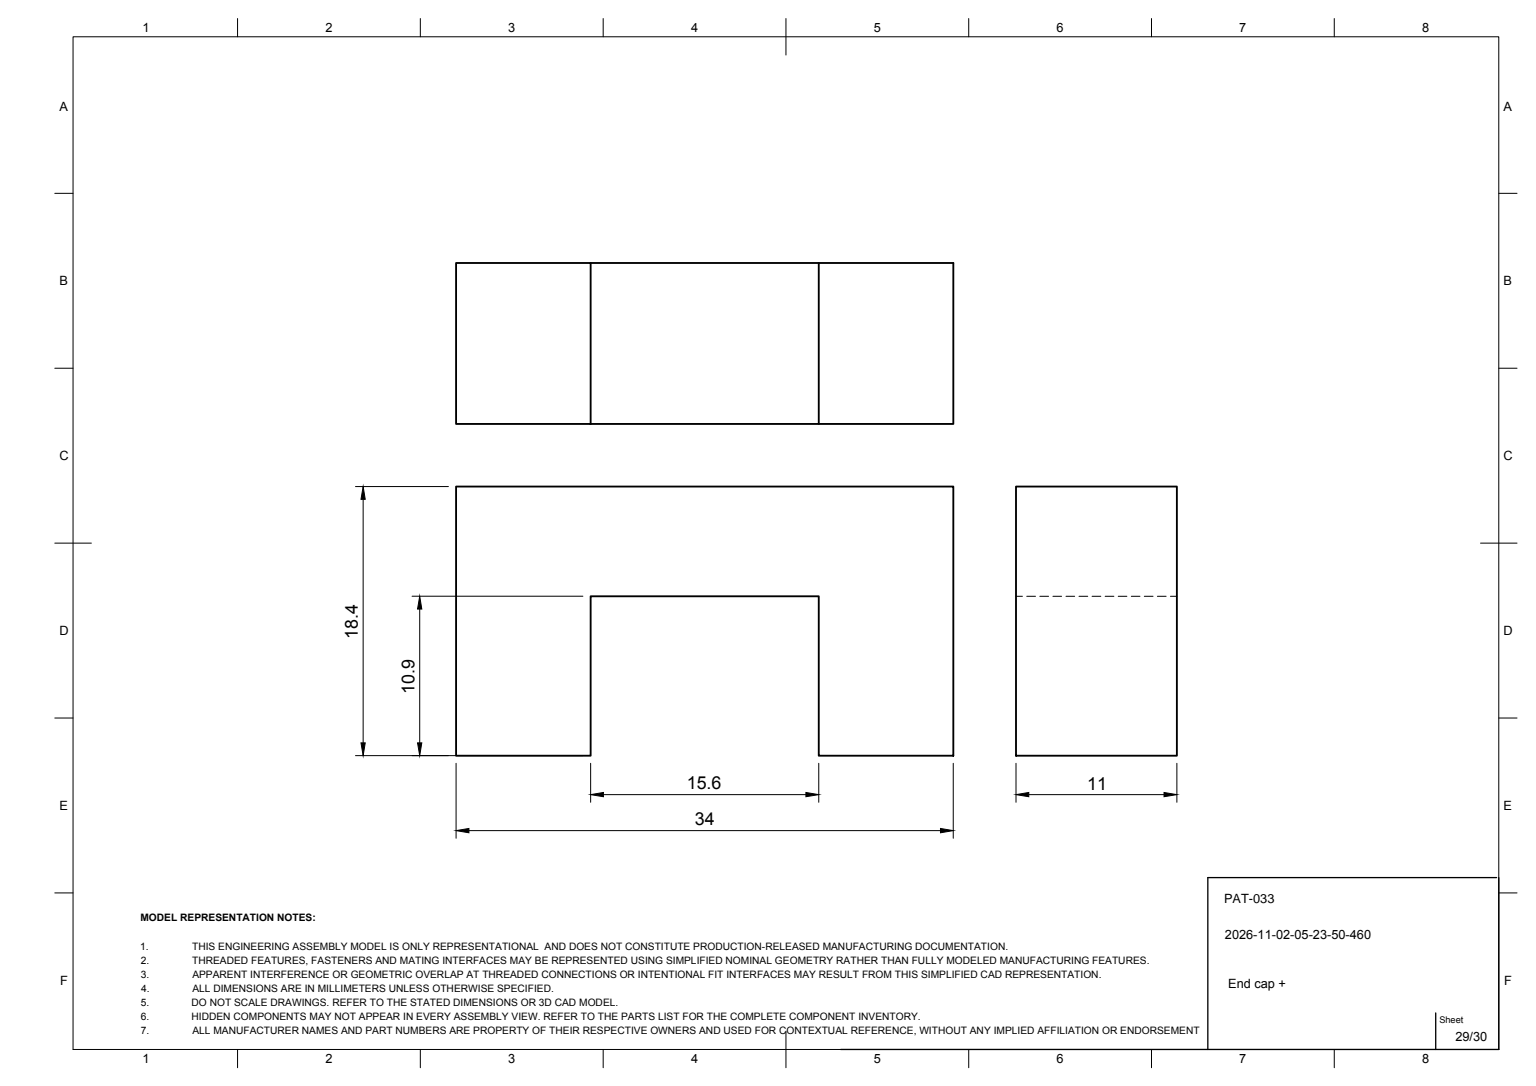
ISO-10303-21;
HEADER;
/* Generated by software containing ST-Developer
 * from STEP Tools, Inc. (www.steptools.com) 
 */

FILE_DESCRIPTION(
/* description */ ('Dual-rail gantry carriage'),
/* implementation_level */ '2;1');

FILE_NAME(
/* name */ 'End cap +.step',
/* time_stamp */ '2026-10-27T10:49:15-07:00',
/* author */ (''),
/* organization */ (''),
/* preprocessor_version */ 'ST-DEVELOPER v20.2',
/* originating_system */ 'Autodesk Translation Framework v15.17.0.0',
/* authorisation */ '');

FILE_SCHEMA (('AUTOMOTIVE_DESIGN { 1 0 10303 214 3 1 1 }'));
ENDSEC;

DATA;
#10=MECHANICAL_DESIGN_GEOMETRIC_PRESENTATION_REPRESENTATION('',(#608),#12804);
#546=SHAPE_REPRESENTATION_RELATIONSHIP('SRR','None',#13026,#577);
#577=ADVANCED_BREP_SHAPE_REPRESENTATION('',(#637),#12796);
#608=STYLED_ITEM('',(#13240),#637);
#637=MANIFOLD_SOLID_BREP('Body1',#7388);
#989=PLANE('',#8239);
#990=PLANE('',#8240);
#991=PLANE('',#8241);
#992=PLANE('',#8242);
#993=PLANE('',#8243);
#994=PLANE('',#8244);
#995=PLANE('',#8245);
#996=PLANE('',#8246);
#997=PLANE('',#8247);
#998=PLANE('',#8248);
#1353=FACE_OUTER_BOUND('',#1855,.T.);
#1354=FACE_OUTER_BOUND('',#1856,.T.);
#1355=FACE_OUTER_BOUND('',#1857,.T.);
#1356=FACE_OUTER_BOUND('',#1858,.T.);
#1357=FACE_OUTER_BOUND('',#1859,.T.);
#1358=FACE_OUTER_BOUND('',#1860,.T.);
#1359=FACE_OUTER_BOUND('',#1861,.T.);
#1360=FACE_OUTER_BOUND('',#1862,.T.);
#1361=FACE_OUTER_BOUND('',#1863,.T.);
#1362=FACE_OUTER_BOUND('',#1864,.T.);
#1855=EDGE_LOOP('',(#6561,#6562,#6563,#6564));
#1856=EDGE_LOOP('',(#6565,#6566,#6567,#6568));
#1857=EDGE_LOOP('',(#6569,#6570,#6571,#6572));
#1858=EDGE_LOOP('',(#6573,#6574,#6575,#6576));
#1859=EDGE_LOOP('',(#6577,#6578,#6579,#6580));
#1860=EDGE_LOOP('',(#6581,#6582,#6583,#6584));
#1861=EDGE_LOOP('',(#6585,#6586,#6587,#6588));
#1862=EDGE_LOOP('',(#6589,#6590,#6591,#6592));
#1863=EDGE_LOOP('',(#6593,#6594,#6595,#6596,#6597,#6598,#6599,#6600));
#1864=EDGE_LOOP('',(#6601,#6602,#6603,#6604,#6605,#6606,#6607,#6608));
#2530=LINE('',#12256,#3239);
#2531=LINE('',#12258,#3240);
#2532=LINE('',#12260,#3241);
#2533=LINE('',#12261,#3242);
#2534=LINE('',#12264,#3243);
#2535=LINE('',#12266,#3244);
#2536=LINE('',#12267,#3245);
#2537=LINE('',#12270,#3246);
#2538=LINE('',#12272,#3247);
#2539=LINE('',#12273,#3248);
#2540=LINE('',#12276,#3249);
#2541=LINE('',#12278,#3250);
#2542=LINE('',#12279,#3251);
#2543=LINE('',#12282,#3252);
#2544=LINE('',#12284,#3253);
#2545=LINE('',#12285,#3254);
#2546=LINE('',#12288,#3255);
#2547=LINE('',#12290,#3256);
#2548=LINE('',#12291,#3257);
#2549=LINE('',#12294,#3258);
#2550=LINE('',#12296,#3259);
#2551=LINE('',#12297,#3260);
#2552=LINE('',#12299,#3261);
#2553=LINE('',#12300,#3262);
#3239=VECTOR('',#10067,1.);
#3240=VECTOR('',#10068,1.);
#3241=VECTOR('',#10069,1.);
#3242=VECTOR('',#10070,1.);
#3243=VECTOR('',#10073,1.);
#3244=VECTOR('',#10074,1.);
#3245=VECTOR('',#10075,1.);
#3246=VECTOR('',#10078,1.);
#3247=VECTOR('',#10079,1.);
#3248=VECTOR('',#10080,1.);
#3249=VECTOR('',#10083,1.);
#3250=VECTOR('',#10084,1.);
#3251=VECTOR('',#10085,1.);
#3252=VECTOR('',#10088,1.);
#3253=VECTOR('',#10089,1.);
#3254=VECTOR('',#10090,1.);
#3255=VECTOR('',#10093,1.);
#3256=VECTOR('',#10094,1.);
#3257=VECTOR('',#10095,1.);
#3258=VECTOR('',#10098,1.);
#3259=VECTOR('',#10099,1.);
#3260=VECTOR('',#10100,1.);
#3261=VECTOR('',#10103,1.);
#3262=VECTOR('',#10104,1.);
#4051=VERTEX_POINT('',#12254);
#4052=VERTEX_POINT('',#12255);
#4053=VERTEX_POINT('',#12257);
#4054=VERTEX_POINT('',#12259);
#4055=VERTEX_POINT('',#12263);
#4056=VERTEX_POINT('',#12265);
#4057=VERTEX_POINT('',#12269);
#4058=VERTEX_POINT('',#12271);
#4059=VERTEX_POINT('',#12275);
#4060=VERTEX_POINT('',#12277);
#4061=VERTEX_POINT('',#12281);
#4062=VERTEX_POINT('',#12283);
#4063=VERTEX_POINT('',#12287);
#4064=VERTEX_POINT('',#12289);
#4065=VERTEX_POINT('',#12293);
#4066=VERTEX_POINT('',#12295);
#4903=EDGE_CURVE('',#4051,#4052,#2530,.T.);
#4904=EDGE_CURVE('',#4052,#4053,#2531,.T.);
#4905=EDGE_CURVE('',#4054,#4053,#2532,.T.);
#4906=EDGE_CURVE('',#4051,#4054,#2533,.T.);
#4907=EDGE_CURVE('',#4055,#4051,#2534,.T.);
#4908=EDGE_CURVE('',#4056,#4054,#2535,.T.);
#4909=EDGE_CURVE('',#4055,#4056,#2536,.T.);
#4910=EDGE_CURVE('',#4057,#4055,#2537,.T.);
#4911=EDGE_CURVE('',#4058,#4056,#2538,.T.);
#4912=EDGE_CURVE('',#4057,#4058,#2539,.T.);
#4913=EDGE_CURVE('',#4059,#4057,#2540,.T.);
#4914=EDGE_CURVE('',#4060,#4058,#2541,.T.);
#4915=EDGE_CURVE('',#4059,#4060,#2542,.T.);
#4916=EDGE_CURVE('',#4061,#4059,#2543,.T.);
#4917=EDGE_CURVE('',#4062,#4060,#2544,.T.);
#4918=EDGE_CURVE('',#4061,#4062,#2545,.T.);
#4919=EDGE_CURVE('',#4063,#4061,#2546,.T.);
#4920=EDGE_CURVE('',#4064,#4062,#2547,.T.);
#4921=EDGE_CURVE('',#4063,#4064,#2548,.T.);
#4922=EDGE_CURVE('',#4065,#4063,#2549,.T.);
#4923=EDGE_CURVE('',#4066,#4064,#2550,.T.);
#4924=EDGE_CURVE('',#4065,#4066,#2551,.T.);
#4925=EDGE_CURVE('',#4052,#4065,#2552,.T.);
#4926=EDGE_CURVE('',#4053,#4066,#2553,.T.);
#6561=ORIENTED_EDGE('',*,*,#4903,.T.);
#6562=ORIENTED_EDGE('',*,*,#4904,.T.);
#6563=ORIENTED_EDGE('',*,*,#4905,.F.);
#6564=ORIENTED_EDGE('',*,*,#4906,.F.);
#6565=ORIENTED_EDGE('',*,*,#4907,.T.);
#6566=ORIENTED_EDGE('',*,*,#4906,.T.);
#6567=ORIENTED_EDGE('',*,*,#4908,.F.);
#6568=ORIENTED_EDGE('',*,*,#4909,.F.);
#6569=ORIENTED_EDGE('',*,*,#4910,.T.);
#6570=ORIENTED_EDGE('',*,*,#4909,.T.);
#6571=ORIENTED_EDGE('',*,*,#4911,.F.);
#6572=ORIENTED_EDGE('',*,*,#4912,.F.);
#6573=ORIENTED_EDGE('',*,*,#4913,.T.);
#6574=ORIENTED_EDGE('',*,*,#4912,.T.);
#6575=ORIENTED_EDGE('',*,*,#4914,.F.);
#6576=ORIENTED_EDGE('',*,*,#4915,.F.);
#6577=ORIENTED_EDGE('',*,*,#4916,.T.);
#6578=ORIENTED_EDGE('',*,*,#4915,.T.);
#6579=ORIENTED_EDGE('',*,*,#4917,.F.);
#6580=ORIENTED_EDGE('',*,*,#4918,.F.);
#6581=ORIENTED_EDGE('',*,*,#4919,.T.);
#6582=ORIENTED_EDGE('',*,*,#4918,.T.);
#6583=ORIENTED_EDGE('',*,*,#4920,.F.);
#6584=ORIENTED_EDGE('',*,*,#4921,.F.);
#6585=ORIENTED_EDGE('',*,*,#4922,.T.);
#6586=ORIENTED_EDGE('',*,*,#4921,.T.);
#6587=ORIENTED_EDGE('',*,*,#4923,.F.);
#6588=ORIENTED_EDGE('',*,*,#4924,.F.);
#6589=ORIENTED_EDGE('',*,*,#4925,.T.);
#6590=ORIENTED_EDGE('',*,*,#4924,.T.);
#6591=ORIENTED_EDGE('',*,*,#4926,.F.);
#6592=ORIENTED_EDGE('',*,*,#4904,.F.);
#6593=ORIENTED_EDGE('',*,*,#4926,.T.);
#6594=ORIENTED_EDGE('',*,*,#4923,.T.);
#6595=ORIENTED_EDGE('',*,*,#4920,.T.);
#6596=ORIENTED_EDGE('',*,*,#4917,.T.);
#6597=ORIENTED_EDGE('',*,*,#4914,.T.);
#6598=ORIENTED_EDGE('',*,*,#4911,.T.);
#6599=ORIENTED_EDGE('',*,*,#4908,.T.);
#6600=ORIENTED_EDGE('',*,*,#4905,.T.);
#6601=ORIENTED_EDGE('',*,*,#4925,.F.);
#6602=ORIENTED_EDGE('',*,*,#4903,.F.);
#6603=ORIENTED_EDGE('',*,*,#4907,.F.);
#6604=ORIENTED_EDGE('',*,*,#4910,.F.);
#6605=ORIENTED_EDGE('',*,*,#4913,.F.);
#6606=ORIENTED_EDGE('',*,*,#4916,.F.);
#6607=ORIENTED_EDGE('',*,*,#4919,.F.);
#6608=ORIENTED_EDGE('',*,*,#4922,.F.);
#7279=ADVANCED_FACE('',(#1353),#989,.T.);
#7280=ADVANCED_FACE('',(#1354),#990,.T.);
#7281=ADVANCED_FACE('',(#1355),#991,.T.);
#7282=ADVANCED_FACE('',(#1356),#992,.T.);
#7283=ADVANCED_FACE('',(#1357),#993,.T.);
#7284=ADVANCED_FACE('',(#1358),#994,.T.);
#7285=ADVANCED_FACE('',(#1359),#995,.T.);
#7286=ADVANCED_FACE('',(#1360),#996,.T.);
#7287=ADVANCED_FACE('',(#1361),#997,.T.);
#7288=ADVANCED_FACE('',(#1362),#998,.F.);
#7388=CLOSED_SHELL('',(#7279,#7280,#7281,#7282,#7283,#7284,#7285,#7286,
#7287,#7288));
#8238=AXIS2_PLACEMENT_3D('',#12252,#10063,#10064);
#8239=AXIS2_PLACEMENT_3D('',#12253,#10065,#10066);
#8240=AXIS2_PLACEMENT_3D('',#12262,#10071,#10072);
#8241=AXIS2_PLACEMENT_3D('',#12268,#10076,#10077);
#8242=AXIS2_PLACEMENT_3D('',#12274,#10081,#10082);
#8243=AXIS2_PLACEMENT_3D('',#12280,#10086,#10087);
#8244=AXIS2_PLACEMENT_3D('',#12286,#10091,#10092);
#8245=AXIS2_PLACEMENT_3D('',#12292,#10096,#10097);
#8246=AXIS2_PLACEMENT_3D('',#12298,#10101,#10102);
#8247=AXIS2_PLACEMENT_3D('',#12301,#10105,#10106);
#8248=AXIS2_PLACEMENT_3D('',#12302,#10107,#10108);
#10063=DIRECTION('axis',(0.,0.,1.));
#10064=DIRECTION('refdir',(1.,0.,0.));
#10065=DIRECTION('center_axis',(0.,0.,1.));
#10066=DIRECTION('ref_axis',(0.,-1.,0.));
#10067=DIRECTION('',(0.,-1.,0.));
#10068=DIRECTION('',(1.,0.,0.));
#10069=DIRECTION('',(0.,-1.,0.));
#10070=DIRECTION('',(1.,0.,0.));
#10071=DIRECTION('center_axis',(0.,1.,0.));
#10072=DIRECTION('ref_axis',(0.,0.,1.));
#10073=DIRECTION('',(0.,0.,1.));
#10074=DIRECTION('',(0.,0.,1.));
#10075=DIRECTION('',(1.,0.,0.));
#10076=DIRECTION('center_axis',(0.,0.,-1.));
#10077=DIRECTION('ref_axis',(0.,1.,0.));
#10078=DIRECTION('',(0.,1.,0.));
#10079=DIRECTION('',(0.,1.,0.));
#10080=DIRECTION('',(1.,0.,0.));
#10081=DIRECTION('center_axis',(0.,-1.,0.));
#10082=DIRECTION('ref_axis',(0.,0.,-1.));
#10083=DIRECTION('',(0.,0.,-1.));
#10084=DIRECTION('',(0.,0.,-1.));
#10085=DIRECTION('',(1.,0.,0.));
#10086=DIRECTION('center_axis',(0.,0.,-1.));
#10087=DIRECTION('ref_axis',(0.,1.,0.));
#10088=DIRECTION('',(0.,1.,0.));
#10089=DIRECTION('',(0.,1.,0.));
#10090=DIRECTION('',(1.,0.,0.));
#10091=DIRECTION('center_axis',(0.,1.,0.));
#10092=DIRECTION('ref_axis',(0.,0.,1.));
#10093=DIRECTION('',(0.,0.,1.));
#10094=DIRECTION('',(0.,0.,1.));
#10095=DIRECTION('',(1.,0.,0.));
#10096=DIRECTION('center_axis',(0.,0.,-1.));
#10097=DIRECTION('ref_axis',(0.,1.,0.));
#10098=DIRECTION('',(0.,1.,0.));
#10099=DIRECTION('',(0.,1.,0.));
#10100=DIRECTION('',(1.,0.,0.));
#10101=DIRECTION('center_axis',(0.,-1.,0.));
#10102=DIRECTION('ref_axis',(0.,0.,-1.));
#10103=DIRECTION('',(0.,0.,-1.));
#10104=DIRECTION('',(0.,0.,-1.));
#10105=DIRECTION('center_axis',(1.,0.,0.));
#10106=DIRECTION('ref_axis',(0.,0.,-1.));
#10107=DIRECTION('center_axis',(1.,0.,0.));
#10108=DIRECTION('ref_axis',(0.,0.,-1.));
#12252=CARTESIAN_POINT('',(0.,0.,0.));
#12253=CARTESIAN_POINT('Origin',(1.97,1.7,2.3));
#12254=CARTESIAN_POINT('',(1.97,1.7,2.3));
#12255=CARTESIAN_POINT('',(1.97,-1.7,2.3));
#12256=CARTESIAN_POINT('',(1.97,1.7,2.3));
#12257=CARTESIAN_POINT('',(3.07,-1.7,2.3));
#12258=CARTESIAN_POINT('',(1.97,-1.7,2.3));
#12259=CARTESIAN_POINT('',(3.07,1.7,2.3));
#12260=CARTESIAN_POINT('',(3.07,1.7,2.3));
#12261=CARTESIAN_POINT('',(1.97,1.7,2.3));
#12262=CARTESIAN_POINT('Origin',(1.97,1.7,0.46));
#12263=CARTESIAN_POINT('',(1.97,1.7,0.46));
#12264=CARTESIAN_POINT('',(1.97,1.7,0.46));
#12265=CARTESIAN_POINT('',(3.07,1.7,0.46));
#12266=CARTESIAN_POINT('',(3.07,1.7,0.46));
#12267=CARTESIAN_POINT('',(1.97,1.7,0.46));
#12268=CARTESIAN_POINT('Origin',(1.97,0.78,0.46));
#12269=CARTESIAN_POINT('',(1.97,0.78,0.46));
#12270=CARTESIAN_POINT('',(1.97,0.78,0.46));
#12271=CARTESIAN_POINT('',(3.07,0.78,0.46));
#12272=CARTESIAN_POINT('',(3.07,0.78,0.46));
#12273=CARTESIAN_POINT('',(1.97,0.78,0.46));
#12274=CARTESIAN_POINT('Origin',(1.97,0.78,1.55));
#12275=CARTESIAN_POINT('',(1.97,0.78,1.55));
#12276=CARTESIAN_POINT('',(1.97,0.78,1.55));
#12277=CARTESIAN_POINT('',(3.07,0.78,1.55));
#12278=CARTESIAN_POINT('',(3.07,0.78,1.55));
#12279=CARTESIAN_POINT('',(1.97,0.78,1.55));
#12280=CARTESIAN_POINT('Origin',(1.97,-0.78,1.55));
#12281=CARTESIAN_POINT('',(1.97,-0.78,1.55));
#12282=CARTESIAN_POINT('',(1.97,-0.78,1.55));
#12283=CARTESIAN_POINT('',(3.07,-0.78,1.55));
#12284=CARTESIAN_POINT('',(3.07,-0.78,1.55));
#12285=CARTESIAN_POINT('',(1.97,-0.78,1.55));
#12286=CARTESIAN_POINT('Origin',(1.97,-0.78,0.46));
#12287=CARTESIAN_POINT('',(1.97,-0.78,0.46));
#12288=CARTESIAN_POINT('',(1.97,-0.78,0.46));
#12289=CARTESIAN_POINT('',(3.07,-0.78,0.46));
#12290=CARTESIAN_POINT('',(3.07,-0.78,0.46));
#12291=CARTESIAN_POINT('',(1.97,-0.78,0.46));
#12292=CARTESIAN_POINT('Origin',(1.97,-1.7,0.46));
#12293=CARTESIAN_POINT('',(1.97,-1.7,0.46));
#12294=CARTESIAN_POINT('',(1.97,-1.7,0.46));
#12295=CARTESIAN_POINT('',(3.07,-1.7,0.46));
#12296=CARTESIAN_POINT('',(3.07,-1.7,0.46));
#12297=CARTESIAN_POINT('',(1.97,-1.7,0.46));
#12298=CARTESIAN_POINT('Origin',(1.97,-1.7,2.3));
#12299=CARTESIAN_POINT('',(1.97,-1.7,2.3));
#12300=CARTESIAN_POINT('',(3.07,-1.7,2.3));
#12301=CARTESIAN_POINT('Origin',(3.07,0.,1.38));
#12302=CARTESIAN_POINT('Origin',(1.97,0.,1.38));
#12760=UNCERTAINTY_MEASURE_WITH_UNIT(LENGTH_MEASURE(0.001),#12805,
'DISTANCE_ACCURACY_VALUE',
'Maximum model space distance between geometric entities at asserted c
onnectivities');
#12768=UNCERTAINTY_MEASURE_WITH_UNIT(LENGTH_MEASURE(0.001),#12805,
'DISTANCE_ACCURACY_VALUE',
'Maximum model space distance between geometric entities at asserted c
onnectivities');
#12796=(
GEOMETRIC_REPRESENTATION_CONTEXT(3)
GLOBAL_UNCERTAINTY_ASSIGNED_CONTEXT((#12760))
GLOBAL_UNIT_ASSIGNED_CONTEXT((#12805,#12807,#12808))
REPRESENTATION_CONTEXT('','3D')
);
#12804=(
GEOMETRIC_REPRESENTATION_CONTEXT(3)
GLOBAL_UNCERTAINTY_ASSIGNED_CONTEXT((#12768))
GLOBAL_UNIT_ASSIGNED_CONTEXT((#12805,#12807,#12808))
REPRESENTATION_CONTEXT('','3D')
);
#12805=(
LENGTH_UNIT()
NAMED_UNIT(*)
SI_UNIT(.CENTI.,.METRE.)
);
#12807=(
NAMED_UNIT(*)
PLANE_ANGLE_UNIT()
SI_UNIT($,.RADIAN.)
);
#12808=(
NAMED_UNIT(*)
SI_UNIT($,.STERADIAN.)
SOLID_ANGLE_UNIT()
);
#12836=SHAPE_DEFINITION_REPRESENTATION(#12871,#13026);
#12871=PRODUCT_DEFINITION_SHAPE('',$,#13062);
#13026=SHAPE_REPRESENTATION('',(#8238),#12796);
#13034=PRODUCT_DEFINITION_CONTEXT('part definition',#13141,'design');
#13062=PRODUCT_DEFINITION('End cap +','End cap +',#13097,#13034);
#13097=PRODUCT_DEFINITION_FORMATION('',$,#13170);
#13141=APPLICATION_CONTEXT(
'Core Data for Automotive Mechanical Design Process');
#13142=PRODUCT_CONTEXT('part definition',#13141,'mechanical');
#13170=PRODUCT('End cap +','End cap +','End cap +',(#13142));
#13234=COLOUR_RGB('Sky Blue',0.24,0.69,0.87);
#13235=FILL_AREA_STYLE_COLOUR('',#13234);
#13236=FILL_AREA_STYLE('',(#13235));
#13237=SURFACE_STYLE_FILL_AREA(#13236);
#13238=SURFACE_SIDE_STYLE('',(#13237));
#13239=SURFACE_STYLE_USAGE(.BOTH.,#13238);
#13240=PRESENTATION_STYLE_ASSIGNMENT((#13239));
ENDSEC;
END-ISO-10303-21;
